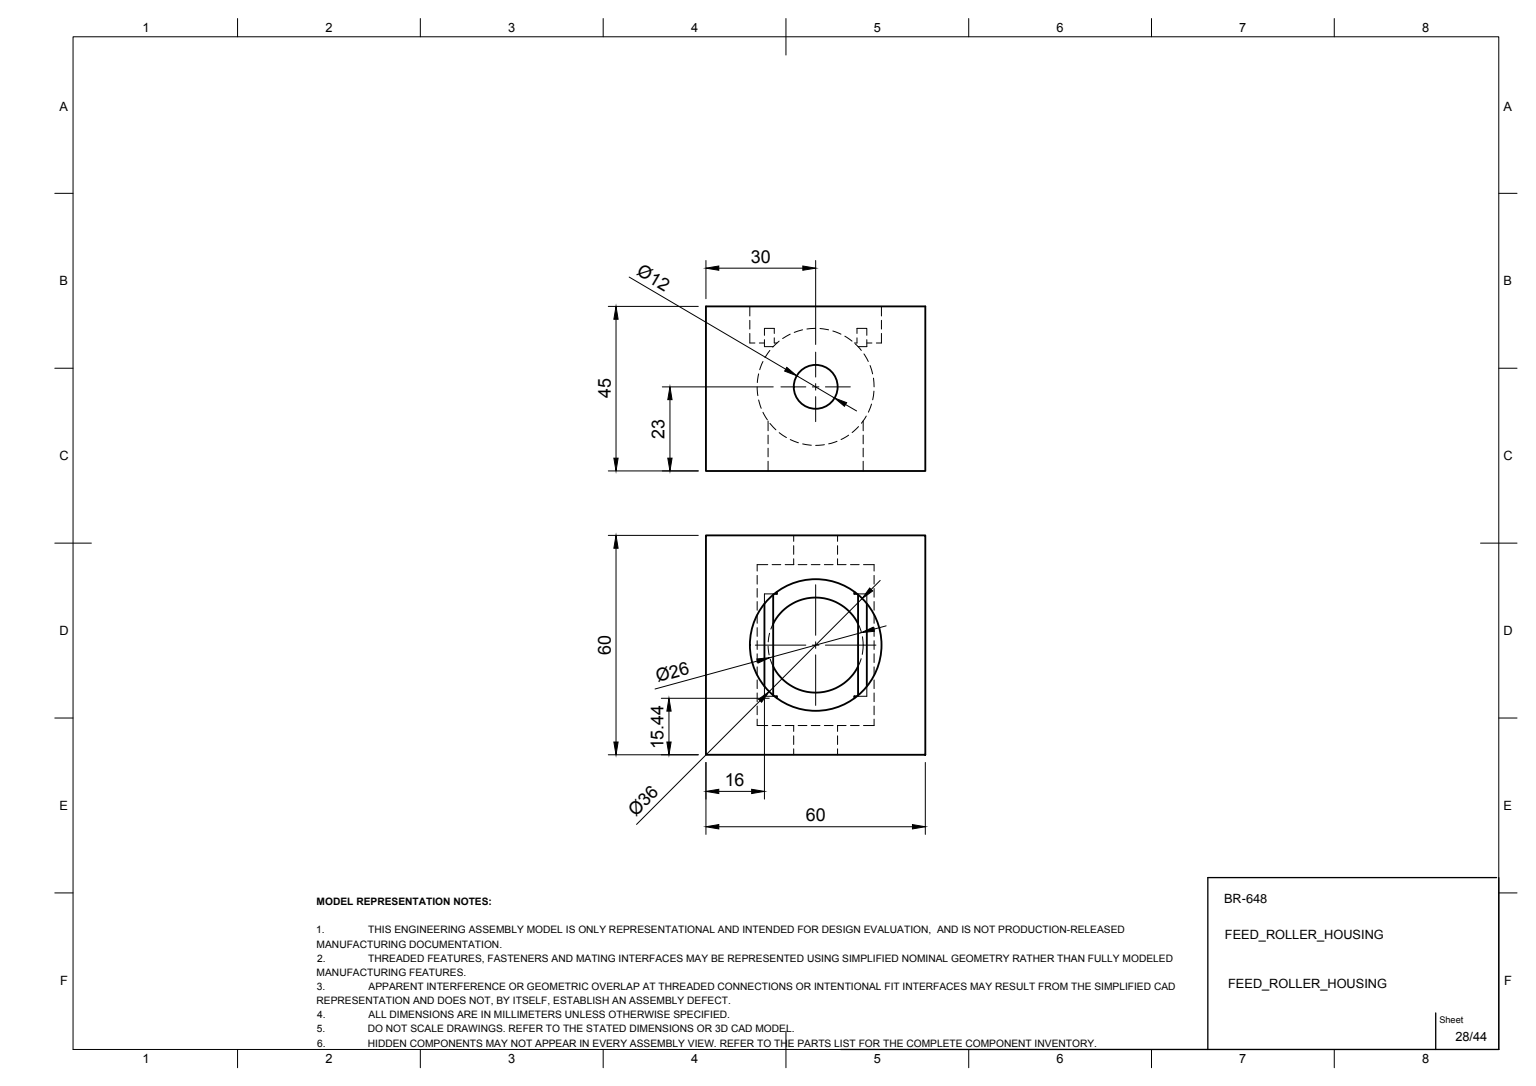
ISO-10303-21;
HEADER;
FILE_DESCRIPTION((''),'2;1');
FILE_NAME('FEED_ROLLER_HOUSING.step','2026-10-01T22:05:39-07:00',(''),(''),'','','');
FILE_SCHEMA (('AUTOMOTIVE_DESIGN { 1 0 10303 214 3 1 1 }'));
ENDSEC;
DATA;
#10=MECHANICAL_DESIGN_GEOMETRIC_PRESENTATION_REPRESENTATION('',(#626),#24628);
#542=SHAPE_REPRESENTATION_RELATIONSHIP('SRR','None',#24815,#584) ;
#584=ADVANCED_BREP_SHAPE_REPRESENTATION('',(#665),#24605) ;
#626=STYLED_ITEM('',(#25031),#665) ;
#665=MANIFOLD_SOLID_BREP('FEED_ROLLER_HOUSING',#13168) ;
#876=FACE_BOUND('',#4451,.T.) ;
#877=FACE_BOUND('',#4452,.T.) ;
#878=FACE_BOUND('',#4454,.T.) ;
#879=FACE_BOUND('',#4456,.T.) ;
#880=FACE_BOUND('',#4460,.T.) ;
#881=FACE_BOUND('',#4462,.T.) ;
#882=FACE_BOUND('',#4464,.T.) ;
#883=FACE_BOUND('',#4467,.T.) ;
#980=B_SPLINE_CURVE_WITH_KNOTS('',3,(#23034,#23035,#23036,#23037,#23038,
#23039,#23040,#23041,#23042,#23043,#23044,#23045,#23046,#23047,#23048,#23049,
#23050,#23051,#23052,#23053,#23054,#23055,#23056,#23057,#23058,#23059),
 .UNSPECIFIED.,.F.,.F.,(4,2,2,2,2,2,2,2,2,2,2,2,4),(0.,0.268031600880283,
0.536063201760566,1.07212640352113,1.58977454134265,1.84859861025342,2.10742267916418,
2.36624674807494,2.6250708169857,3.14271895480722,3.67878215656779,3.94681375744807,
4.21484535832835),.UNSPECIFIED.) ;
#981=B_SPLINE_CURVE_WITH_KNOTS('',3,(#23060,#23061,#23062,#23063,#23064,
#23065,#23066,#23067,#23068,#23069,#23070,#23071,#23072,#23073,#23074,#23075,
#23076,#23077,#23078,#23079,#23080,#23081,#23082,#23083,#23084,#23085),
 .UNSPECIFIED.,.F.,.F.,(4,2,2,2,2,2,2,2,2,2,2,2,4),(4.21484535832835,4.48287695920864,
4.75090856008892,5.28697176184949,5.80461989967101,6.06344396858177,6.32226803749253,
6.58109210640329,6.83991617531405,7.35756431313557,7.89362751489614,8.16165911577642,
8.42969071665671),.UNSPECIFIED.) ;
#982=B_SPLINE_CURVE_WITH_KNOTS('',3,(#23105,#23106,#23107,#23108,#23109,
#23110,#23111,#23112,#23113,#23114,#23115,#23116,#23117,#23118,#23119,#23120,
#23121,#23122),.UNSPECIFIED.,.F.,.F.,(4,2,2,2,2,2,2,2,4),(6.84192042814915,
7.05142392525706,7.37435159053249,7.69727925580792,8.02020692108334,8.34313458635877,
8.6660622516342,8.98898991690963,9.19849341401755),.UNSPECIFIED.) ;
#983=B_SPLINE_CURVE_WITH_KNOTS('',3,(#23124,#23125,#23126,#23127,#23128,
#23129,#23130,#23131,#23132,#23133,#23134,#23135,#23136,#23137,#23138,#23139,
#23140,#23141),.UNSPECIFIED.,.F.,.F.,(4,2,2,2,2,2,2,2,4),(1.49511581409358,
1.7046193112015,2.02754697647693,2.35047464175235,2.67340230702778,2.99632997230321,
3.31925763757864,3.64218530285406,3.85168879996198),.UNSPECIFIED.) ;
#1487=LINE('',#22927,#2323) ;
#1488=LINE('',#22929,#2324) ;
#1489=LINE('',#22931,#2325) ;
#1490=LINE('',#22933,#2326) ;
#1491=LINE('',#22935,#2327) ;
#1492=LINE('',#22937,#2328) ;
#1493=LINE('',#22939,#2329) ;
#1494=LINE('',#22940,#2330) ;
#1495=LINE('',#22944,#2331) ;
#1496=LINE('',#22946,#2332) ;
#1497=LINE('',#22948,#2333) ;
#1498=LINE('',#22949,#2334) ;
#1499=LINE('',#22954,#2335) ;
#1500=LINE('',#22956,#2336) ;
#1501=LINE('',#22958,#2337) ;
#1502=LINE('',#22959,#2338) ;
#1503=LINE('',#22964,#2339) ;
#1504=LINE('',#22966,#2340) ;
#1505=LINE('',#22968,#2341) ;
#1506=LINE('',#22969,#2342) ;
#1507=LINE('',#22973,#2343) ;
#1508=LINE('',#22974,#2344) ;
#1509=LINE('',#22976,#2345) ;
#1510=LINE('',#22979,#2346) ;
#1511=LINE('',#22983,#2347) ;
#1512=LINE('',#22989,#2348) ;
#1513=LINE('',#22993,#2349) ;
#1514=LINE('',#22996,#2350) ;
#1515=LINE('',#22997,#2351) ;
#1516=LINE('',#23000,#2352) ;
#1517=LINE('',#23002,#2353) ;
#1518=LINE('',#23006,#2354) ;
#1519=LINE('',#23008,#2355) ;
#1520=LINE('',#23009,#2356) ;
#1521=LINE('',#23012,#2357) ;
#1522=LINE('',#23017,#2358) ;
#1523=LINE('',#23025,#2359) ;
#1524=LINE('',#23032,#2360) ;
#1525=LINE('',#23090,#2361) ;
#1526=LINE('',#23096,#2362) ;
#1527=LINE('',#23102,#2363) ;
#1528=LINE('',#23123,#2364) ;
#1529=LINE('',#23148,#2365) ;
#1530=LINE('',#23153,#2366) ;
#1531=LINE('',#23155,#2367) ;
#1532=LINE('',#23157,#2368) ;
#1533=LINE('',#23158,#2369) ;
#1534=LINE('',#23162,#2370) ;
#1535=LINE('',#23164,#2371) ;
#1536=LINE('',#23166,#2372) ;
#1537=LINE('',#23167,#2373) ;
#1538=LINE('',#23169,#2374) ;
#1539=LINE('',#23170,#2375) ;
#1540=LINE('',#23172,#2376) ;
#1541=LINE('',#23174,#2377) ;
#2323=VECTOR('',#18344,1.) ;
#2324=VECTOR('',#18345,1.) ;
#2325=VECTOR('',#18346,1.) ;
#2326=VECTOR('',#18347,1.) ;
#2327=VECTOR('',#18348,1.) ;
#2328=VECTOR('',#18349,1.) ;
#2329=VECTOR('',#18350,1.) ;
#2330=VECTOR('',#18351,1.) ;
#2331=VECTOR('',#18354,1.) ;
#2332=VECTOR('',#18355,1.) ;
#2333=VECTOR('',#18356,1.) ;
#2334=VECTOR('',#18357,1.) ;
#2335=VECTOR('',#18362,1.) ;
#2336=VECTOR('',#18363,1.) ;
#2337=VECTOR('',#18364,1.) ;
#2338=VECTOR('',#18365,1.) ;
#2339=VECTOR('',#18370,1.) ;
#2340=VECTOR('',#18371,1.) ;
#2341=VECTOR('',#18372,1.) ;
#2342=VECTOR('',#18373,1.) ;
#2343=VECTOR('',#18376,1.) ;
#2344=VECTOR('',#18377,1.) ;
#2345=VECTOR('',#18378,1.) ;
#2346=VECTOR('',#18381,1.) ;
#2347=VECTOR('',#18386,1.) ;
#2348=VECTOR('',#18395,1.) ;
#2349=VECTOR('',#18400,1.) ;
#2350=VECTOR('',#18403,1.) ;
#2351=VECTOR('',#18404,1.) ;
#2352=VECTOR('',#18407,1.) ;
#2353=VECTOR('',#18408,1.) ;
#2354=VECTOR('',#18413,1.) ;
#2355=VECTOR('',#18414,1.) ;
#2356=VECTOR('',#18415,1.) ;
#2357=VECTOR('',#18418,1.) ;
#2358=VECTOR('',#18425,1.) ;
#2359=VECTOR('',#18436,1.) ;
#2360=VECTOR('',#18445,1.3) ;
#2361=VECTOR('',#18450,0.6) ;
#2362=VECTOR('',#18457,0.6) ;
#2363=VECTOR('',#18464,1.6) ;
#2364=VECTOR('',#18467,1.) ;
#2365=VECTOR('',#18478,1.8) ;
#2366=VECTOR('',#18483,1.) ;
#2367=VECTOR('',#18484,1.) ;
#2368=VECTOR('',#18485,1.) ;
#2369=VECTOR('',#18486,1.) ;
#2370=VECTOR('',#18489,1.) ;
#2371=VECTOR('',#18490,1.) ;
#2372=VECTOR('',#18491,1.) ;
#2373=VECTOR('',#18492,1.) ;
#2374=VECTOR('',#18495,1.) ;
#2375=VECTOR('',#18496,1.) ;
#2376=VECTOR('',#18499,1.) ;
#2377=VECTOR('',#18502,1.) ;
#2875=CYLINDRICAL_SURFACE('',#14916,1.3) ;
#2876=CYLINDRICAL_SURFACE('',#14918,0.6) ;
#2877=CYLINDRICAL_SURFACE('',#14921,0.6) ;
#2878=CYLINDRICAL_SURFACE('',#14924,1.6) ;
#2879=CYLINDRICAL_SURFACE('',#14931,1.8) ;
#3473=FACE_OUTER_BOUND('',#4430,.T.) ;
#3474=FACE_OUTER_BOUND('',#4431,.T.) ;
#3475=FACE_OUTER_BOUND('',#4432,.T.) ;
#3476=FACE_OUTER_BOUND('',#4433,.T.) ;
#3477=FACE_OUTER_BOUND('',#4434,.T.) ;
#3478=FACE_OUTER_BOUND('',#4435,.T.) ;
#3479=FACE_OUTER_BOUND('',#4436,.T.) ;
#3480=FACE_OUTER_BOUND('',#4437,.T.) ;
#3481=FACE_OUTER_BOUND('',#4438,.T.) ;
#3482=FACE_OUTER_BOUND('',#4439,.T.) ;
#3483=FACE_OUTER_BOUND('',#4440,.T.) ;
#3484=FACE_OUTER_BOUND('',#4441,.T.) ;
#3485=FACE_OUTER_BOUND('',#4442,.T.) ;
#3486=FACE_OUTER_BOUND('',#4443,.T.) ;
#3487=FACE_OUTER_BOUND('',#4444,.T.) ;
#3488=FACE_OUTER_BOUND('',#4445,.T.) ;
#3489=FACE_OUTER_BOUND('',#4446,.T.) ;
#3490=FACE_OUTER_BOUND('',#4447,.T.) ;
#3491=FACE_OUTER_BOUND('',#4448,.T.) ;
#3492=FACE_OUTER_BOUND('',#4449,.T.) ;
#3493=FACE_OUTER_BOUND('',#4450,.T.) ;
#3494=FACE_OUTER_BOUND('',#4453,.T.) ;
#3495=FACE_OUTER_BOUND('',#4455,.T.) ;
#3496=FACE_OUTER_BOUND('',#4457,.T.) ;
#3497=FACE_OUTER_BOUND('',#4458,.T.) ;
#3498=FACE_OUTER_BOUND('',#4459,.T.) ;
#3499=FACE_OUTER_BOUND('',#4461,.T.) ;
#3500=FACE_OUTER_BOUND('',#4463,.T.) ;
#3501=FACE_OUTER_BOUND('',#4465,.T.) ;
#3502=FACE_OUTER_BOUND('',#4466,.T.) ;
#3503=FACE_OUTER_BOUND('',#4468,.T.) ;
#4430=EDGE_LOOP('',(#10863,#10864,#10865,#10866,#10867,#10868,#10869,#10870)) ;
#4431=EDGE_LOOP('',(#10871,#10872,#10873,#10874)) ;
#4432=EDGE_LOOP('',(#10875,#10876,#10877,#10878,#10879,#10880)) ;
#4433=EDGE_LOOP('',(#10881,#10882,#10883,#10884,#10885,#10886)) ;
#4434=EDGE_LOOP('',(#10887,#10888,#10889,#10890,#10891,#10892)) ;
#4435=EDGE_LOOP('',(#10893,#10894,#10895)) ;
#4436=EDGE_LOOP('',(#10896,#10897,#10898)) ;
#4437=EDGE_LOOP('',(#10899,#10900,#10901)) ;
#4438=EDGE_LOOP('',(#10902,#10903,#10904)) ;
#4439=EDGE_LOOP('',(#10905,#10906,#10907,#10908)) ;
#4440=EDGE_LOOP('',(#10909,#10910,#10911,#10912,#10913,#10914)) ;
#4441=EDGE_LOOP('',(#10915,#10916,#10917,#10918,#10919,#10920,#10921,#10922)) ;
#4442=EDGE_LOOP('',(#10923,#10924,#10925)) ;
#4443=EDGE_LOOP('',(#10926,#10927,#10928)) ;
#4444=EDGE_LOOP('',(#10929,#10930,#10931)) ;
#4445=EDGE_LOOP('',(#10932,#10933,#10934)) ;
#4446=EDGE_LOOP('',(#10935,#10936)) ;
#4447=EDGE_LOOP('',(#10937,#10938,#10939,#10940,#10941)) ;
#4448=EDGE_LOOP('',(#10942,#10943,#10944,#10945)) ;
#4449=EDGE_LOOP('',(#10946,#10947,#10948,#10949)) ;
#4450=EDGE_LOOP('',(#10950,#10951,#10952,#10953)) ;
#4451=EDGE_LOOP('',(#10954,#10955,#10956,#10957,#10958,#10959,#10960,#10961,
#10962,#10963,#10964,#10965)) ;
#4452=EDGE_LOOP('',(#10966,#10967)) ;
#4453=EDGE_LOOP('',(#10968)) ;
#4454=EDGE_LOOP('',(#10969)) ;
#4455=EDGE_LOOP('',(#10970)) ;
#4456=EDGE_LOOP('',(#10971)) ;
#4457=EDGE_LOOP('',(#10972,#10973,#10974)) ;
#4458=EDGE_LOOP('',(#10975,#10976,#10977,#10978,#10979,#10980,#10981,#10982,
#10983,#10984,#10985,#10986,#10987,#10988,#10989,#10990,#10991,#10992,#10993,
#10994,#10995,#10996,#10997,#10998)) ;
#4459=EDGE_LOOP('',(#10999,#11000,#11001,#11002)) ;
#4460=EDGE_LOOP('',(#11003)) ;
#4461=EDGE_LOOP('',(#11004,#11005,#11006,#11007)) ;
#4462=EDGE_LOOP('',(#11008)) ;
#4463=EDGE_LOOP('',(#11009,#11010,#11011,#11012)) ;
#4464=EDGE_LOOP('',(#11013)) ;
#4465=EDGE_LOOP('',(#11014,#11015,#11016,#11017)) ;
#4466=EDGE_LOOP('',(#11018,#11019,#11020,#11021)) ;
#4467=EDGE_LOOP('',(#11022)) ;
#4468=EDGE_LOOP('',(#11023,#11024,#11025,#11026)) ;
#5348=CIRCLE('',#14888,1.6) ;
#5349=CIRCLE('',#14890,1.6) ;
#5350=CIRCLE('',#14892,1.6) ;
#5351=CIRCLE('',#14894,1.8) ;
#5352=CIRCLE('',#14896,1.8) ;
#5353=CIRCLE('',#14898,1.8) ;
#5354=CIRCLE('',#14900,1.8) ;
#5355=CIRCLE('',#14903,1.6) ;
#5356=CIRCLE('',#14906,1.8) ;
#5357=CIRCLE('',#14908,1.8) ;
#5358=CIRCLE('',#14910,1.8) ;
#5359=CIRCLE('',#14911,1.8) ;
#5360=CIRCLE('',#14913,1.8) ;
#5361=CIRCLE('',#14915,1.8) ;
#5362=CIRCLE('',#14917,1.3) ;
#5363=CIRCLE('',#14919,0.6) ;
#5364=CIRCLE('',#14920,0.6) ;
#5365=CIRCLE('',#14922,0.6) ;
#5366=CIRCLE('',#14923,0.6) ;
#5367=CIRCLE('',#14925,1.6) ;
#5368=CIRCLE('',#14926,1.6) ;
#5369=CIRCLE('',#14930,1.8) ;
#5370=CIRCLE('',#14932,1.8) ;
#6358=VERTEX_POINT('',#22925) ;
#6359=VERTEX_POINT('',#22926) ;
#6360=VERTEX_POINT('',#22928) ;
#6361=VERTEX_POINT('',#22930) ;
#6362=VERTEX_POINT('',#22932) ;
#6363=VERTEX_POINT('',#22934) ;
#6364=VERTEX_POINT('',#22936) ;
#6365=VERTEX_POINT('',#22938) ;
#6366=VERTEX_POINT('',#22942) ;
#6367=VERTEX_POINT('',#22943) ;
#6368=VERTEX_POINT('',#22945) ;
#6369=VERTEX_POINT('',#22947) ;
#6370=VERTEX_POINT('',#22951) ;
#6371=VERTEX_POINT('',#22953) ;
#6372=VERTEX_POINT('',#22955) ;
#6373=VERTEX_POINT('',#22957) ;
#6374=VERTEX_POINT('',#22961) ;
#6375=VERTEX_POINT('',#22963) ;
#6376=VERTEX_POINT('',#22965) ;
#6377=VERTEX_POINT('',#22967) ;
#6378=VERTEX_POINT('',#22971) ;
#6379=VERTEX_POINT('',#22972) ;
#6380=VERTEX_POINT('',#22975) ;
#6381=VERTEX_POINT('',#22977) ;
#6382=VERTEX_POINT('',#22981) ;
#6383=VERTEX_POINT('',#22987) ;
#6384=VERTEX_POINT('',#22991) ;
#6385=VERTEX_POINT('',#22995) ;
#6386=VERTEX_POINT('',#22999) ;
#6387=VERTEX_POINT('',#23001) ;
#6388=VERTEX_POINT('',#23005) ;
#6389=VERTEX_POINT('',#23007) ;
#6390=VERTEX_POINT('',#23011) ;
#6391=VERTEX_POINT('',#23015) ;
#6392=VERTEX_POINT('',#23019) ;
#6393=VERTEX_POINT('',#23023) ;
#6394=VERTEX_POINT('',#23029) ;
#6395=VERTEX_POINT('',#23031) ;
#6396=VERTEX_POINT('',#23033) ;
#6397=VERTEX_POINT('',#23087) ;
#6398=VERTEX_POINT('',#23089) ;
#6399=VERTEX_POINT('',#23093) ;
#6400=VERTEX_POINT('',#23095) ;
#6401=VERTEX_POINT('',#23099) ;
#6402=VERTEX_POINT('',#23101) ;
#6403=VERTEX_POINT('',#23104) ;
#6404=VERTEX_POINT('',#23147) ;
#6405=VERTEX_POINT('',#23151) ;
#6406=VERTEX_POINT('',#23152) ;
#6407=VERTEX_POINT('',#23154) ;
#6408=VERTEX_POINT('',#23156) ;
#6409=VERTEX_POINT('',#23160) ;
#6410=VERTEX_POINT('',#23161) ;
#6411=VERTEX_POINT('',#23163) ;
#6412=VERTEX_POINT('',#23165) ;
#7921=EDGE_CURVE('',#6358,#6359,#1487,.T.) ;
#7922=EDGE_CURVE('',#6358,#6360,#1488,.T.) ;
#7923=EDGE_CURVE('',#6360,#6361,#1489,.T.) ;
#7924=EDGE_CURVE('',#6361,#6362,#1490,.T.) ;
#7925=EDGE_CURVE('',#6363,#6362,#1491,.T.) ;
#7926=EDGE_CURVE('',#6363,#6364,#1492,.T.) ;
#7927=EDGE_CURVE('',#6365,#6364,#1493,.T.) ;
#7928=EDGE_CURVE('',#6359,#6365,#1494,.T.) ;
#7929=EDGE_CURVE('',#6366,#6367,#1495,.T.) ;
#7930=EDGE_CURVE('',#6368,#6366,#1496,.T.) ;
#7931=EDGE_CURVE('',#6369,#6368,#1497,.T.) ;
#7932=EDGE_CURVE('',#6367,#6369,#1498,.T.) ;
#7933=EDGE_CURVE('',#6370,#6366,#5348,.T.) ;
#7934=EDGE_CURVE('',#6371,#6370,#1499,.T.) ;
#7935=EDGE_CURVE('',#6372,#6371,#1500,.T.) ;
#7936=EDGE_CURVE('',#6372,#6373,#1501,.T.) ;
#7937=EDGE_CURVE('',#6373,#6368,#1502,.T.) ;
#7938=EDGE_CURVE('',#6367,#6374,#5349,.T.) ;
#7939=EDGE_CURVE('',#6375,#6369,#1503,.T.) ;
#7940=EDGE_CURVE('',#6375,#6376,#1504,.T.) ;
#7941=EDGE_CURVE('',#6377,#6376,#1505,.T.) ;
#7942=EDGE_CURVE('',#6374,#6377,#1506,.T.) ;
#7943=EDGE_CURVE('',#6378,#6379,#1507,.T.) ;
#7944=EDGE_CURVE('',#6378,#6363,#1508,.T.) ;
#7945=EDGE_CURVE('',#6362,#6380,#1509,.T.) ;
#7946=EDGE_CURVE('',#6381,#6380,#5350,.T.) ;
#7947=EDGE_CURVE('',#6379,#6381,#1510,.T.) ;
#7948=EDGE_CURVE('',#6376,#6382,#5351,.T.) ;
#7949=EDGE_CURVE('',#6382,#6375,#1511,.T.) ;
#7950=EDGE_CURVE('',#6364,#6378,#5352,.T.) ;
#7951=EDGE_CURVE('',#6383,#6372,#5353,.T.) ;
#7952=EDGE_CURVE('',#6373,#6383,#1512,.T.) ;
#7953=EDGE_CURVE('',#6384,#6358,#5354,.T.) ;
#7954=EDGE_CURVE('',#6360,#6384,#1513,.T.) ;
#7955=EDGE_CURVE('',#6380,#6385,#1514,.T.) ;
#7956=EDGE_CURVE('',#6385,#6361,#1515,.T.) ;
#7957=EDGE_CURVE('',#6386,#6384,#1516,.T.) ;
#7958=EDGE_CURVE('',#6387,#6386,#1517,.T.) ;
#7959=EDGE_CURVE('',#6385,#6387,#5355,.T.) ;
#7960=EDGE_CURVE('',#6388,#6383,#1518,.T.) ;
#7961=EDGE_CURVE('',#6389,#6388,#1519,.T.) ;
#7962=EDGE_CURVE('',#6382,#6389,#1520,.T.) ;
#7963=EDGE_CURVE('',#6381,#6390,#1521,.T.) ;
#7964=EDGE_CURVE('',#6379,#6390,#5356,.T.) ;
#7965=EDGE_CURVE('',#6391,#6386,#5357,.T.) ;
#7966=EDGE_CURVE('',#6391,#6387,#1522,.T.) ;
#7967=EDGE_CURVE('',#6392,#6365,#5358,.T.) ;
#7968=EDGE_CURVE('',#6359,#6392,#5359,.T.) ;
#7969=EDGE_CURVE('',#6393,#6377,#5360,.T.) ;
#7970=EDGE_CURVE('',#6393,#6374,#1523,.T.) ;
#7971=EDGE_CURVE('',#6389,#6388,#5361,.T.) ;
#7972=EDGE_CURVE('',#6394,#6394,#5362,.T.) ;
#7973=EDGE_CURVE('',#6394,#6395,#1524,.T.) ;
#7974=EDGE_CURVE('',#6396,#6395,#980,.T.) ;
#7975=EDGE_CURVE('',#6395,#6396,#981,.T.) ;
#7976=EDGE_CURVE('',#6397,#6397,#5363,.T.) ;
#7977=EDGE_CURVE('',#6397,#6398,#1525,.T.) ;
#7978=EDGE_CURVE('',#6398,#6398,#5364,.T.) ;
#7979=EDGE_CURVE('',#6399,#6399,#5365,.T.) ;
#7980=EDGE_CURVE('',#6399,#6400,#1526,.T.) ;
#7981=EDGE_CURVE('',#6400,#6400,#5366,.T.) ;
#7982=EDGE_CURVE('',#6401,#6401,#5367,.T.) ;
#7983=EDGE_CURVE('',#6401,#6402,#1527,.T.) ;
#7984=EDGE_CURVE('',#6402,#6402,#5368,.T.) ;
#7985=EDGE_CURVE('',#6403,#6391,#982,.T.) ;
#7986=EDGE_CURVE('',#6370,#6403,#1528,.T.) ;
#7987=EDGE_CURVE('',#6390,#6393,#983,.T.) ;
#7988=EDGE_CURVE('',#6371,#6403,#5369,.T.) ;
#7989=EDGE_CURVE('',#6392,#6404,#1529,.T.) ;
#7990=EDGE_CURVE('',#6404,#6404,#5370,.T.) ;
#7991=EDGE_CURVE('',#6405,#6406,#1530,.T.) ;
#7992=EDGE_CURVE('',#6406,#6407,#1531,.T.) ;
#7993=EDGE_CURVE('',#6407,#6408,#1532,.T.) ;
#7994=EDGE_CURVE('',#6408,#6405,#1533,.T.) ;
#7995=EDGE_CURVE('',#6409,#6410,#1534,.T.) ;
#7996=EDGE_CURVE('',#6410,#6411,#1535,.T.) ;
#7997=EDGE_CURVE('',#6411,#6412,#1536,.T.) ;
#7998=EDGE_CURVE('',#6412,#6409,#1537,.T.) ;
#7999=EDGE_CURVE('',#6408,#6411,#1538,.T.) ;
#8000=EDGE_CURVE('',#6405,#6410,#1539,.T.) ;
#8001=EDGE_CURVE('',#6407,#6412,#1540,.T.) ;
#8002=EDGE_CURVE('',#6406,#6409,#1541,.T.) ;
#10863=ORIENTED_EDGE('',*,*,#7921,.F.) ;
#10864=ORIENTED_EDGE('',*,*,#7922,.T.) ;
#10865=ORIENTED_EDGE('',*,*,#7923,.T.) ;
#10866=ORIENTED_EDGE('',*,*,#7924,.T.) ;
#10867=ORIENTED_EDGE('',*,*,#7925,.F.) ;
#10868=ORIENTED_EDGE('',*,*,#7926,.T.) ;
#10869=ORIENTED_EDGE('',*,*,#7927,.F.) ;
#10870=ORIENTED_EDGE('',*,*,#7928,.F.) ;
#10871=ORIENTED_EDGE('',*,*,#7929,.F.) ;
#10872=ORIENTED_EDGE('',*,*,#7930,.F.) ;
#10873=ORIENTED_EDGE('',*,*,#7931,.F.) ;
#10874=ORIENTED_EDGE('',*,*,#7932,.F.) ;
#10875=ORIENTED_EDGE('',*,*,#7933,.F.) ;
#10876=ORIENTED_EDGE('',*,*,#7934,.F.) ;
#10877=ORIENTED_EDGE('',*,*,#7935,.F.) ;
#10878=ORIENTED_EDGE('',*,*,#7936,.T.) ;
#10879=ORIENTED_EDGE('',*,*,#7937,.T.) ;
#10880=ORIENTED_EDGE('',*,*,#7930,.T.) ;
#10881=ORIENTED_EDGE('',*,*,#7938,.F.) ;
#10882=ORIENTED_EDGE('',*,*,#7932,.T.) ;
#10883=ORIENTED_EDGE('',*,*,#7939,.F.) ;
#10884=ORIENTED_EDGE('',*,*,#7940,.T.) ;
#10885=ORIENTED_EDGE('',*,*,#7941,.F.) ;
#10886=ORIENTED_EDGE('',*,*,#7942,.F.) ;
#10887=ORIENTED_EDGE('',*,*,#7943,.F.) ;
#10888=ORIENTED_EDGE('',*,*,#7944,.T.) ;
#10889=ORIENTED_EDGE('',*,*,#7925,.T.) ;
#10890=ORIENTED_EDGE('',*,*,#7945,.T.) ;
#10891=ORIENTED_EDGE('',*,*,#7946,.F.) ;
#10892=ORIENTED_EDGE('',*,*,#7947,.F.) ;
#10893=ORIENTED_EDGE('',*,*,#7948,.F.) ;
#10894=ORIENTED_EDGE('',*,*,#7940,.F.) ;
#10895=ORIENTED_EDGE('',*,*,#7949,.F.) ;
#10896=ORIENTED_EDGE('',*,*,#7950,.F.) ;
#10897=ORIENTED_EDGE('',*,*,#7926,.F.) ;
#10898=ORIENTED_EDGE('',*,*,#7944,.F.) ;
#10899=ORIENTED_EDGE('',*,*,#7951,.F.) ;
#10900=ORIENTED_EDGE('',*,*,#7952,.F.) ;
#10901=ORIENTED_EDGE('',*,*,#7936,.F.) ;
#10902=ORIENTED_EDGE('',*,*,#7953,.F.) ;
#10903=ORIENTED_EDGE('',*,*,#7954,.F.) ;
#10904=ORIENTED_EDGE('',*,*,#7922,.F.) ;
#10905=ORIENTED_EDGE('',*,*,#7955,.F.) ;
#10906=ORIENTED_EDGE('',*,*,#7945,.F.) ;
#10907=ORIENTED_EDGE('',*,*,#7924,.F.) ;
#10908=ORIENTED_EDGE('',*,*,#7956,.F.) ;
#10909=ORIENTED_EDGE('',*,*,#7957,.F.) ;
#10910=ORIENTED_EDGE('',*,*,#7958,.F.) ;
#10911=ORIENTED_EDGE('',*,*,#7959,.F.) ;
#10912=ORIENTED_EDGE('',*,*,#7956,.T.) ;
#10913=ORIENTED_EDGE('',*,*,#7923,.F.) ;
#10914=ORIENTED_EDGE('',*,*,#7954,.T.) ;
#10915=ORIENTED_EDGE('',*,*,#7960,.F.) ;
#10916=ORIENTED_EDGE('',*,*,#7961,.F.) ;
#10917=ORIENTED_EDGE('',*,*,#7962,.F.) ;
#10918=ORIENTED_EDGE('',*,*,#7949,.T.) ;
#10919=ORIENTED_EDGE('',*,*,#7939,.T.) ;
#10920=ORIENTED_EDGE('',*,*,#7931,.T.) ;
#10921=ORIENTED_EDGE('',*,*,#7937,.F.) ;
#10922=ORIENTED_EDGE('',*,*,#7952,.T.) ;
#10923=ORIENTED_EDGE('',*,*,#7947,.T.) ;
#10924=ORIENTED_EDGE('',*,*,#7963,.T.) ;
#10925=ORIENTED_EDGE('',*,*,#7964,.F.) ;
#10926=ORIENTED_EDGE('',*,*,#7958,.T.) ;
#10927=ORIENTED_EDGE('',*,*,#7965,.F.) ;
#10928=ORIENTED_EDGE('',*,*,#7966,.T.) ;
#10929=ORIENTED_EDGE('',*,*,#7928,.T.) ;
#10930=ORIENTED_EDGE('',*,*,#7967,.F.) ;
#10931=ORIENTED_EDGE('',*,*,#7968,.F.) ;
#10932=ORIENTED_EDGE('',*,*,#7942,.T.) ;
#10933=ORIENTED_EDGE('',*,*,#7969,.F.) ;
#10934=ORIENTED_EDGE('',*,*,#7970,.T.) ;
#10935=ORIENTED_EDGE('',*,*,#7961,.T.) ;
#10936=ORIENTED_EDGE('',*,*,#7971,.F.) ;
#10937=ORIENTED_EDGE('',*,*,#7972,.F.) ;
#10938=ORIENTED_EDGE('',*,*,#7973,.T.) ;
#10939=ORIENTED_EDGE('',*,*,#7974,.F.) ;
#10940=ORIENTED_EDGE('',*,*,#7975,.F.) ;
#10941=ORIENTED_EDGE('',*,*,#7973,.F.) ;
#10942=ORIENTED_EDGE('',*,*,#7976,.F.) ;
#10943=ORIENTED_EDGE('',*,*,#7977,.T.) ;
#10944=ORIENTED_EDGE('',*,*,#7978,.F.) ;
#10945=ORIENTED_EDGE('',*,*,#7977,.F.) ;
#10946=ORIENTED_EDGE('',*,*,#7979,.F.) ;
#10947=ORIENTED_EDGE('',*,*,#7980,.T.) ;
#10948=ORIENTED_EDGE('',*,*,#7981,.F.) ;
#10949=ORIENTED_EDGE('',*,*,#7980,.F.) ;
#10950=ORIENTED_EDGE('',*,*,#7982,.T.) ;
#10951=ORIENTED_EDGE('',*,*,#7983,.T.) ;
#10952=ORIENTED_EDGE('',*,*,#7984,.T.) ;
#10953=ORIENTED_EDGE('',*,*,#7983,.F.) ;
#10954=ORIENTED_EDGE('',*,*,#7959,.T.) ;
#10955=ORIENTED_EDGE('',*,*,#7966,.F.) ;
#10956=ORIENTED_EDGE('',*,*,#7985,.F.) ;
#10957=ORIENTED_EDGE('',*,*,#7986,.F.) ;
#10958=ORIENTED_EDGE('',*,*,#7933,.T.) ;
#10959=ORIENTED_EDGE('',*,*,#7929,.T.) ;
#10960=ORIENTED_EDGE('',*,*,#7938,.T.) ;
#10961=ORIENTED_EDGE('',*,*,#7970,.F.) ;
#10962=ORIENTED_EDGE('',*,*,#7987,.F.) ;
#10963=ORIENTED_EDGE('',*,*,#7963,.F.) ;
#10964=ORIENTED_EDGE('',*,*,#7946,.T.) ;
#10965=ORIENTED_EDGE('',*,*,#7955,.T.) ;
#10966=ORIENTED_EDGE('',*,*,#7974,.T.) ;
#10967=ORIENTED_EDGE('',*,*,#7975,.T.) ;
#10968=ORIENTED_EDGE('',*,*,#7982,.F.) ;
#10969=ORIENTED_EDGE('',*,*,#7981,.T.) ;
#10970=ORIENTED_EDGE('',*,*,#7984,.F.) ;
#10971=ORIENTED_EDGE('',*,*,#7976,.T.) ;
#10972=ORIENTED_EDGE('',*,*,#7934,.T.) ;
#10973=ORIENTED_EDGE('',*,*,#7986,.T.) ;
#10974=ORIENTED_EDGE('',*,*,#7988,.F.) ;
#10975=ORIENTED_EDGE('',*,*,#7921,.T.) ;
#10976=ORIENTED_EDGE('',*,*,#7968,.T.) ;
#10977=ORIENTED_EDGE('',*,*,#7989,.T.) ;
#10978=ORIENTED_EDGE('',*,*,#7990,.F.) ;
#10979=ORIENTED_EDGE('',*,*,#7989,.F.) ;
#10980=ORIENTED_EDGE('',*,*,#7967,.T.) ;
#10981=ORIENTED_EDGE('',*,*,#7927,.T.) ;
#10982=ORIENTED_EDGE('',*,*,#7950,.T.) ;
#10983=ORIENTED_EDGE('',*,*,#7943,.T.) ;
#10984=ORIENTED_EDGE('',*,*,#7964,.T.) ;
#10985=ORIENTED_EDGE('',*,*,#7987,.T.) ;
#10986=ORIENTED_EDGE('',*,*,#7969,.T.) ;
#10987=ORIENTED_EDGE('',*,*,#7941,.T.) ;
#10988=ORIENTED_EDGE('',*,*,#7948,.T.) ;
#10989=ORIENTED_EDGE('',*,*,#7962,.T.) ;
#10990=ORIENTED_EDGE('',*,*,#7971,.T.) ;
#10991=ORIENTED_EDGE('',*,*,#7960,.T.) ;
#10992=ORIENTED_EDGE('',*,*,#7951,.T.) ;
#10993=ORIENTED_EDGE('',*,*,#7935,.T.) ;
#10994=ORIENTED_EDGE('',*,*,#7988,.T.) ;
#10995=ORIENTED_EDGE('',*,*,#7985,.T.) ;
#10996=ORIENTED_EDGE('',*,*,#7965,.T.) ;
#10997=ORIENTED_EDGE('',*,*,#7957,.T.) ;
#10998=ORIENTED_EDGE('',*,*,#7953,.T.) ;
#10999=ORIENTED_EDGE('',*,*,#7991,.T.) ;
#11000=ORIENTED_EDGE('',*,*,#7992,.T.) ;
#11001=ORIENTED_EDGE('',*,*,#7993,.T.) ;
#11002=ORIENTED_EDGE('',*,*,#7994,.T.) ;
#11003=ORIENTED_EDGE('',*,*,#7990,.T.) ;
#11004=ORIENTED_EDGE('',*,*,#7995,.T.) ;
#11005=ORIENTED_EDGE('',*,*,#7996,.T.) ;
#11006=ORIENTED_EDGE('',*,*,#7997,.T.) ;
#11007=ORIENTED_EDGE('',*,*,#7998,.T.) ;
#11008=ORIENTED_EDGE('',*,*,#7972,.T.) ;
#11009=ORIENTED_EDGE('',*,*,#7999,.T.) ;
#11010=ORIENTED_EDGE('',*,*,#7996,.F.) ;
#11011=ORIENTED_EDGE('',*,*,#8000,.F.) ;
#11012=ORIENTED_EDGE('',*,*,#7994,.F.) ;
#11013=ORIENTED_EDGE('',*,*,#7979,.T.) ;
#11014=ORIENTED_EDGE('',*,*,#8001,.T.) ;
#11015=ORIENTED_EDGE('',*,*,#7997,.F.) ;
#11016=ORIENTED_EDGE('',*,*,#7999,.F.) ;
#11017=ORIENTED_EDGE('',*,*,#7993,.F.) ;
#11018=ORIENTED_EDGE('',*,*,#8002,.T.) ;
#11019=ORIENTED_EDGE('',*,*,#7998,.F.) ;
#11020=ORIENTED_EDGE('',*,*,#8001,.F.) ;
#11021=ORIENTED_EDGE('',*,*,#7992,.F.) ;
#11022=ORIENTED_EDGE('',*,*,#7978,.T.) ;
#11023=ORIENTED_EDGE('',*,*,#8000,.T.) ;
#11024=ORIENTED_EDGE('',*,*,#7995,.F.) ;
#11025=ORIENTED_EDGE('',*,*,#8002,.F.) ;
#11026=ORIENTED_EDGE('',*,*,#7991,.F.) ;
#12183=PLANE('',#14885) ;
#12184=PLANE('',#14886) ;
#12185=PLANE('',#14887) ;
#12186=PLANE('',#14889) ;
#12187=PLANE('',#14891) ;
#12188=PLANE('',#14893) ;
#12189=PLANE('',#14895) ;
#12190=PLANE('',#14897) ;
#12191=PLANE('',#14899) ;
#12192=PLANE('',#14901) ;
#12193=PLANE('',#14902) ;
#12194=PLANE('',#14904) ;
#12195=PLANE('',#14905) ;
#12196=PLANE('',#14907) ;
#12197=PLANE('',#14909) ;
#12198=PLANE('',#14912) ;
#12199=PLANE('',#14914) ;
#12200=PLANE('',#14927) ;
#12201=PLANE('',#14928) ;
#12202=PLANE('',#14929) ;
#12203=PLANE('',#14933) ;
#12204=PLANE('',#14934) ;
#12205=PLANE('',#14935) ;
#12206=PLANE('',#14936) ;
#12207=PLANE('',#14937) ;
#12208=PLANE('',#14938) ;
#12868=ADVANCED_FACE('',(#3473),#12183,.T.) ;
#12869=ADVANCED_FACE('',(#3474),#12184,.T.) ;
#12870=ADVANCED_FACE('',(#3475),#12185,.T.) ;
#12871=ADVANCED_FACE('',(#3476),#12186,.T.) ;
#12872=ADVANCED_FACE('',(#3477),#12187,.T.) ;
#12873=ADVANCED_FACE('',(#3478),#12188,.F.) ;
#12874=ADVANCED_FACE('',(#3479),#12189,.F.) ;
#12875=ADVANCED_FACE('',(#3480),#12190,.F.) ;
#12876=ADVANCED_FACE('',(#3481),#12191,.F.) ;
#12877=ADVANCED_FACE('',(#3482),#12192,.T.) ;
#12878=ADVANCED_FACE('',(#3483),#12193,.T.) ;
#12879=ADVANCED_FACE('',(#3484),#12194,.T.) ;
#12880=ADVANCED_FACE('',(#3485),#12195,.F.) ;
#12881=ADVANCED_FACE('',(#3486),#12196,.F.) ;
#12882=ADVANCED_FACE('',(#3487),#12197,.F.) ;
#12883=ADVANCED_FACE('',(#3488),#12198,.F.) ;
#12884=ADVANCED_FACE('',(#3489),#12199,.F.) ;
#12885=ADVANCED_FACE('',(#3490),#2875,.F.) ;
#12886=ADVANCED_FACE('',(#3491),#2876,.F.) ;
#12887=ADVANCED_FACE('',(#3492),#2877,.F.) ;
#12888=ADVANCED_FACE('',(#3493,#876,#877),#2878,.F.) ;
#12889=ADVANCED_FACE('',(#3494,#878),#12200,.F.) ;
#12890=ADVANCED_FACE('',(#3495,#879),#12201,.F.) ;
#12891=ADVANCED_FACE('',(#3496),#12202,.F.) ;
#12892=ADVANCED_FACE('',(#3497),#2879,.F.) ;
#12893=ADVANCED_FACE('',(#3498,#880),#12203,.T.) ;
#12894=ADVANCED_FACE('',(#3499,#881),#12204,.F.) ;
#12895=ADVANCED_FACE('',(#3500,#882),#12205,.F.) ;
#12896=ADVANCED_FACE('',(#3501),#12206,.F.) ;
#12897=ADVANCED_FACE('',(#3502,#883),#12207,.F.) ;
#12898=ADVANCED_FACE('',(#3503),#12208,.F.) ;
#13168=CLOSED_SHELL('',(#12868,#12869,#12870,#12871,#12872,#12873,#12874,
#12875,#12876,#12877,#12878,#12879,#12880,#12881,#12882,#12883,#12884,#12885,
#12886,#12887,#12888,#12889,#12890,#12891,#12892,#12893,#12894,#12895,#12896,
#12897,#12898)) ;
#14884=AXIS2_PLACEMENT_3D('',#22923,#18340,#18341) ;
#14885=AXIS2_PLACEMENT_3D('',#22924,#18342,#18343) ;
#14886=AXIS2_PLACEMENT_3D('',#22941,#18352,#18353) ;
#14887=AXIS2_PLACEMENT_3D('',#22950,#18358,#18359) ;
#14888=AXIS2_PLACEMENT_3D('',#22952,#18360,#18361) ;
#14889=AXIS2_PLACEMENT_3D('',#22960,#18366,#18367) ;
#14890=AXIS2_PLACEMENT_3D('',#22962,#18368,#18369) ;
#14891=AXIS2_PLACEMENT_3D('',#22970,#18374,#18375) ;
#14892=AXIS2_PLACEMENT_3D('',#22978,#18379,#18380) ;
#14893=AXIS2_PLACEMENT_3D('',#22980,#18382,#18383) ;
#14894=AXIS2_PLACEMENT_3D('',#22982,#18384,#18385) ;
#14895=AXIS2_PLACEMENT_3D('',#22984,#18387,#18388) ;
#14896=AXIS2_PLACEMENT_3D('',#22985,#18389,#18390) ;
#14897=AXIS2_PLACEMENT_3D('',#22986,#18391,#18392) ;
#14898=AXIS2_PLACEMENT_3D('',#22988,#18393,#18394) ;
#14899=AXIS2_PLACEMENT_3D('',#22990,#18396,#18397) ;
#14900=AXIS2_PLACEMENT_3D('',#22992,#18398,#18399) ;
#14901=AXIS2_PLACEMENT_3D('',#22994,#18401,#18402) ;
#14902=AXIS2_PLACEMENT_3D('',#22998,#18405,#18406) ;
#14903=AXIS2_PLACEMENT_3D('',#23003,#18409,#18410) ;
#14904=AXIS2_PLACEMENT_3D('',#23004,#18411,#18412) ;
#14905=AXIS2_PLACEMENT_3D('',#23010,#18416,#18417) ;
#14906=AXIS2_PLACEMENT_3D('',#23013,#18419,#18420) ;
#14907=AXIS2_PLACEMENT_3D('',#23014,#18421,#18422) ;
#14908=AXIS2_PLACEMENT_3D('',#23016,#18423,#18424) ;
#14909=AXIS2_PLACEMENT_3D('',#23018,#18426,#18427) ;
#14910=AXIS2_PLACEMENT_3D('',#23020,#18428,#18429) ;
#14911=AXIS2_PLACEMENT_3D('',#23021,#18430,#18431) ;
#14912=AXIS2_PLACEMENT_3D('',#23022,#18432,#18433) ;
#14913=AXIS2_PLACEMENT_3D('',#23024,#18434,#18435) ;
#14914=AXIS2_PLACEMENT_3D('',#23026,#18437,#18438) ;
#14915=AXIS2_PLACEMENT_3D('',#23027,#18439,#18440) ;
#14916=AXIS2_PLACEMENT_3D('',#23028,#18441,#18442) ;
#14917=AXIS2_PLACEMENT_3D('',#23030,#18443,#18444) ;
#14918=AXIS2_PLACEMENT_3D('',#23086,#18446,#18447) ;
#14919=AXIS2_PLACEMENT_3D('',#23088,#18448,#18449) ;
#14920=AXIS2_PLACEMENT_3D('',#23091,#18451,#18452) ;
#14921=AXIS2_PLACEMENT_3D('',#23092,#18453,#18454) ;
#14922=AXIS2_PLACEMENT_3D('',#23094,#18455,#18456) ;
#14923=AXIS2_PLACEMENT_3D('',#23097,#18458,#18459) ;
#14924=AXIS2_PLACEMENT_3D('',#23098,#18460,#18461) ;
#14925=AXIS2_PLACEMENT_3D('',#23100,#18462,#18463) ;
#14926=AXIS2_PLACEMENT_3D('',#23103,#18465,#18466) ;
#14927=AXIS2_PLACEMENT_3D('',#23142,#18468,#18469) ;
#14928=AXIS2_PLACEMENT_3D('',#23143,#18470,#18471) ;
#14929=AXIS2_PLACEMENT_3D('',#23144,#18472,#18473) ;
#14930=AXIS2_PLACEMENT_3D('',#23145,#18474,#18475) ;
#14931=AXIS2_PLACEMENT_3D('',#23146,#18476,#18477) ;
#14932=AXIS2_PLACEMENT_3D('',#23149,#18479,#18480) ;
#14933=AXIS2_PLACEMENT_3D('',#23150,#18481,#18482) ;
#14934=AXIS2_PLACEMENT_3D('',#23159,#18487,#18488) ;
#14935=AXIS2_PLACEMENT_3D('',#23168,#18493,#18494) ;
#14936=AXIS2_PLACEMENT_3D('',#23171,#18497,#18498) ;
#14937=AXIS2_PLACEMENT_3D('',#23173,#18500,#18501) ;
#14938=AXIS2_PLACEMENT_3D('',#23175,#18503,#18504) ;
#18340=DIRECTION('axis',(0.,0.,1.)) ;
#18341=DIRECTION('refdir',(1.,0.,0.)) ;
#18342=DIRECTION('center_axis',(1.,0.,0.)) ;
#18343=DIRECTION('ref_axis',(0.,0.,-1.)) ;
#18344=DIRECTION('',(0.,0.,-1.)) ;
#18345=DIRECTION('',(0.,-1.,0.)) ;
#18346=DIRECTION('',(0.,0.,-1.)) ;
#18347=DIRECTION('',(0.,1.,0.)) ;
#18348=DIRECTION('',(0.,0.,-1.)) ;
#18349=DIRECTION('',(0.,-1.,0.)) ;
#18350=DIRECTION('',(0.,0.,1.)) ;
#18351=DIRECTION('',(0.,1.,0.)) ;
#18352=DIRECTION('center_axis',(0.,0.,1.)) ;
#18353=DIRECTION('ref_axis',(1.,0.,0.)) ;
#18354=DIRECTION('',(0.,1.,0.)) ;
#18355=DIRECTION('',(-1.,0.,0.)) ;
#18356=DIRECTION('',(0.,-1.,0.)) ;
#18357=DIRECTION('',(1.,0.,0.)) ;
#18358=DIRECTION('center_axis',(0.,1.,0.)) ;
#18359=DIRECTION('ref_axis',(0.,0.,1.)) ;
#18360=DIRECTION('center_axis',(0.,1.,0.)) ;
#18361=DIRECTION('ref_axis',(1.,0.,0.)) ;
#18362=DIRECTION('',(-1.,0.,0.)) ;
#18363=DIRECTION('',(0.,0.,-1.)) ;
#18364=DIRECTION('',(1.,0.,0.)) ;
#18365=DIRECTION('',(0.,0.,-1.)) ;
#18366=DIRECTION('center_axis',(0.,-1.,0.)) ;
#18367=DIRECTION('ref_axis',(0.,0.,-1.)) ;
#18368=DIRECTION('center_axis',(0.,-1.,0.)) ;
#18369=DIRECTION('ref_axis',(1.,0.,0.)) ;
#18370=DIRECTION('',(0.,0.,-1.)) ;
#18371=DIRECTION('',(-1.,0.,0.)) ;
#18372=DIRECTION('',(0.,0.,1.)) ;
#18373=DIRECTION('',(1.,0.,0.)) ;
#18374=DIRECTION('center_axis',(0.,-1.,0.)) ;
#18375=DIRECTION('ref_axis',(0.,0.,-1.)) ;
#18376=DIRECTION('',(0.,0.,-1.)) ;
#18377=DIRECTION('',(-1.,0.,0.)) ;
#18378=DIRECTION('',(1.,0.,0.)) ;
#18379=DIRECTION('center_axis',(0.,-1.,0.)) ;
#18380=DIRECTION('ref_axis',(1.,0.,0.)) ;
#18381=DIRECTION('',(1.,0.,0.)) ;
#18382=DIRECTION('center_axis',(0.,0.,1.)) ;
#18383=DIRECTION('ref_axis',(1.,0.,0.)) ;
#18384=DIRECTION('center_axis',(0.,0.,-1.)) ;
#18385=DIRECTION('ref_axis',(1.,0.,0.)) ;
#18386=DIRECTION('',(0.,1.,0.)) ;
#18387=DIRECTION('center_axis',(0.,0.,1.)) ;
#18388=DIRECTION('ref_axis',(1.,0.,0.)) ;
#18389=DIRECTION('center_axis',(0.,0.,-1.)) ;
#18390=DIRECTION('ref_axis',(1.,0.,0.)) ;
#18391=DIRECTION('center_axis',(0.,0.,1.)) ;
#18392=DIRECTION('ref_axis',(1.,0.,0.)) ;
#18393=DIRECTION('center_axis',(0.,0.,-1.)) ;
#18394=DIRECTION('ref_axis',(1.,0.,0.)) ;
#18395=DIRECTION('',(0.,1.,0.)) ;
#18396=DIRECTION('center_axis',(0.,0.,1.)) ;
#18397=DIRECTION('ref_axis',(1.,0.,0.)) ;
#18398=DIRECTION('center_axis',(0.,0.,-1.)) ;
#18399=DIRECTION('ref_axis',(1.,0.,0.)) ;
#18400=DIRECTION('',(1.,0.,0.)) ;
#18401=DIRECTION('center_axis',(0.,0.,1.)) ;
#18402=DIRECTION('ref_axis',(1.,0.,0.)) ;
#18403=DIRECTION('',(0.,-1.,0.)) ;
#18404=DIRECTION('',(-1.,0.,0.)) ;
#18405=DIRECTION('center_axis',(0.,1.,0.)) ;
#18406=DIRECTION('ref_axis',(0.,0.,1.)) ;
#18407=DIRECTION('',(0.,0.,1.)) ;
#18408=DIRECTION('',(-1.,0.,0.)) ;
#18409=DIRECTION('center_axis',(0.,1.,0.)) ;
#18410=DIRECTION('ref_axis',(1.,0.,0.)) ;
#18411=DIRECTION('center_axis',(-1.,0.,0.)) ;
#18412=DIRECTION('ref_axis',(0.,0.,1.)) ;
#18413=DIRECTION('',(0.,0.,1.)) ;
#18414=DIRECTION('',(0.,-1.,0.)) ;
#18415=DIRECTION('',(0.,0.,-1.)) ;
#18416=DIRECTION('center_axis',(0.,0.,-1.)) ;
#18417=DIRECTION('ref_axis',(-1.,0.,0.)) ;
#18418=DIRECTION('',(0.,1.,0.)) ;
#18419=DIRECTION('center_axis',(0.,0.,-1.)) ;
#18420=DIRECTION('ref_axis',(1.,0.,0.)) ;
#18421=DIRECTION('center_axis',(0.,0.,-1.)) ;
#18422=DIRECTION('ref_axis',(-1.,0.,0.)) ;
#18423=DIRECTION('center_axis',(0.,0.,-1.)) ;
#18424=DIRECTION('ref_axis',(1.,0.,0.)) ;
#18425=DIRECTION('',(0.,1.,0.)) ;
#18426=DIRECTION('center_axis',(0.,0.,-1.)) ;
#18427=DIRECTION('ref_axis',(-1.,0.,0.)) ;
#18428=DIRECTION('center_axis',(0.,0.,-1.)) ;
#18429=DIRECTION('ref_axis',(1.,0.,0.)) ;
#18430=DIRECTION('center_axis',(0.,0.,-1.)) ;
#18431=DIRECTION('ref_axis',(1.,0.,0.)) ;
#18432=DIRECTION('center_axis',(0.,0.,-1.)) ;
#18433=DIRECTION('ref_axis',(-1.,0.,0.)) ;
#18434=DIRECTION('center_axis',(0.,0.,-1.)) ;
#18435=DIRECTION('ref_axis',(1.,0.,0.)) ;
#18436=DIRECTION('',(0.,-1.,0.)) ;
#18437=DIRECTION('center_axis',(0.,0.,-1.)) ;
#18438=DIRECTION('ref_axis',(-1.,0.,0.)) ;
#18439=DIRECTION('center_axis',(0.,0.,-1.)) ;
#18440=DIRECTION('ref_axis',(1.,0.,0.)) ;
#18441=DIRECTION('center_axis',(0.,0.,1.)) ;
#18442=DIRECTION('ref_axis',(1.,0.,0.)) ;
#18443=DIRECTION('center_axis',(0.,0.,1.)) ;
#18444=DIRECTION('ref_axis',(1.,0.,0.)) ;
#18445=DIRECTION('',(0.,0.,1.)) ;
#18446=DIRECTION('center_axis',(0.,1.,0.)) ;
#18447=DIRECTION('ref_axis',(1.,0.,0.)) ;
#18448=DIRECTION('center_axis',(0.,1.,0.)) ;
#18449=DIRECTION('ref_axis',(1.,0.,0.)) ;
#18450=DIRECTION('',(0.,1.,0.)) ;
#18451=DIRECTION('center_axis',(0.,-1.,0.)) ;
#18452=DIRECTION('ref_axis',(1.,0.,0.)) ;
#18453=DIRECTION('center_axis',(0.,1.,0.)) ;
#18454=DIRECTION('ref_axis',(1.,0.,0.)) ;
#18455=DIRECTION('center_axis',(0.,1.,0.)) ;
#18456=DIRECTION('ref_axis',(1.,0.,0.)) ;
#18457=DIRECTION('',(0.,1.,0.)) ;
#18458=DIRECTION('center_axis',(0.,-1.,0.)) ;
#18459=DIRECTION('ref_axis',(1.,0.,0.)) ;
#18460=DIRECTION('center_axis',(0.,1.,0.)) ;
#18461=DIRECTION('ref_axis',(1.,0.,0.)) ;
#18462=DIRECTION('center_axis',(0.,-1.,0.)) ;
#18463=DIRECTION('ref_axis',(1.,0.,0.)) ;
#18464=DIRECTION('',(0.,1.,0.)) ;
#18465=DIRECTION('center_axis',(0.,1.,0.)) ;
#18466=DIRECTION('ref_axis',(1.,0.,0.)) ;
#18467=DIRECTION('',(0.,-1.,0.)) ;
#18468=DIRECTION('center_axis',(0.,-1.,0.)) ;
#18469=DIRECTION('ref_axis',(-1.,0.,0.)) ;
#18470=DIRECTION('center_axis',(0.,1.,0.)) ;
#18471=DIRECTION('ref_axis',(1.,0.,0.)) ;
#18472=DIRECTION('center_axis',(0.,0.,-1.)) ;
#18473=DIRECTION('ref_axis',(-1.,0.,0.)) ;
#18474=DIRECTION('center_axis',(0.,0.,-1.)) ;
#18475=DIRECTION('ref_axis',(1.,0.,0.)) ;
#18476=DIRECTION('center_axis',(0.,0.,1.)) ;
#18477=DIRECTION('ref_axis',(1.,0.,0.)) ;
#18478=DIRECTION('',(0.,0.,1.)) ;
#18479=DIRECTION('center_axis',(0.,0.,-1.)) ;
#18480=DIRECTION('ref_axis',(1.,0.,0.)) ;
#18481=DIRECTION('center_axis',(0.,0.,1.)) ;
#18482=DIRECTION('ref_axis',(1.,0.,0.)) ;
#18483=DIRECTION('',(0.,1.,0.)) ;
#18484=DIRECTION('',(-1.,0.,0.)) ;
#18485=DIRECTION('',(0.,-1.,0.)) ;
#18486=DIRECTION('',(1.,0.,0.)) ;
#18487=DIRECTION('center_axis',(0.,0.,1.)) ;
#18488=DIRECTION('ref_axis',(1.,0.,0.)) ;
#18489=DIRECTION('',(0.,-1.,0.)) ;
#18490=DIRECTION('',(-1.,0.,0.)) ;
#18491=DIRECTION('',(0.,1.,0.)) ;
#18492=DIRECTION('',(1.,0.,0.)) ;
#18493=DIRECTION('center_axis',(0.,1.,0.)) ;
#18494=DIRECTION('ref_axis',(0.,0.,1.)) ;
#18495=DIRECTION('',(0.,0.,-1.)) ;
#18496=DIRECTION('',(0.,0.,-1.)) ;
#18497=DIRECTION('center_axis',(1.,0.,0.)) ;
#18498=DIRECTION('ref_axis',(0.,0.,-1.)) ;
#18499=DIRECTION('',(0.,0.,-1.)) ;
#18500=DIRECTION('center_axis',(0.,-1.,0.)) ;
#18501=DIRECTION('ref_axis',(0.,0.,-1.)) ;
#18502=DIRECTION('',(0.,0.,-1.)) ;
#18503=DIRECTION('center_axis',(-1.,0.,0.)) ;
#18504=DIRECTION('ref_axis',(0.,0.,1.)) ;
#22923=CARTESIAN_POINT('',(0.,0.,0.)) ;
#22924=CARTESIAN_POINT('Origin',(-24.4,-1.8,-0.85)) ;
#22925=CARTESIAN_POINT('',(-24.4,-2.93137084989848,-0.6)) ;
#22926=CARTESIAN_POINT('',(-24.4,-2.93137084989848,-1.)) ;
#22927=CARTESIAN_POINT('',(-24.4,-2.93137084989848,-0.45)) ;
#22928=CARTESIAN_POINT('',(-24.4,-3.2,-0.6)) ;
#22929=CARTESIAN_POINT('',(-24.4,-1.8,-0.6)) ;
#22930=CARTESIAN_POINT('',(-24.4,-3.2,-1.1)) ;
#22931=CARTESIAN_POINT('',(-24.4,-3.2,-0.85)) ;
#22932=CARTESIAN_POINT('',(-24.4,-0.4,-1.1)) ;
#22933=CARTESIAN_POINT('',(-24.4,-1.8,-1.1)) ;
#22934=CARTESIAN_POINT('',(-24.4,-0.4,-0.6)) ;
#22935=CARTESIAN_POINT('',(-24.4,-0.4,-0.85)) ;
#22936=CARTESIAN_POINT('',(-24.4,-0.668629150101522,-0.6)) ;
#22937=CARTESIAN_POINT('',(-24.4,-1.8,-0.6)) ;
#22938=CARTESIAN_POINT('',(-24.4,-0.668629150101522,-1.)) ;
#22939=CARTESIAN_POINT('',(-24.4,-0.668629150101522,-0.45)) ;
#22940=CARTESIAN_POINT('',(-24.4,-1.8,-1.)) ;
#22941=CARTESIAN_POINT('Origin',(-23.,-1.8,-1.1)) ;
#22942=CARTESIAN_POINT('',(-21.8381049961378,-3.2,-1.1)) ;
#22943=CARTESIAN_POINT('',(-21.8381049961378,-0.4,-1.1)) ;
#22944=CARTESIAN_POINT('',(-21.8381049961378,-1.8,-1.1)) ;
#22945=CARTESIAN_POINT('',(-21.6,-3.2,-1.1)) ;
#22946=CARTESIAN_POINT('',(-23.,-3.2,-1.1)) ;
#22947=CARTESIAN_POINT('',(-21.6,-0.4,-1.1)) ;
#22948=CARTESIAN_POINT('',(-21.6,-1.8,-1.1)) ;
#22949=CARTESIAN_POINT('',(-23.,-0.4,-1.1)) ;
#22950=CARTESIAN_POINT('Origin',(-23.,-3.2,-0.85)) ;
#22951=CARTESIAN_POINT('',(-21.9416994755742,-3.2,-1.)) ;
#22952=CARTESIAN_POINT('Origin',(-23.,-3.2,-2.2)) ;
#22953=CARTESIAN_POINT('',(-21.8686291501015,-3.2,-1.)) ;
#22954=CARTESIAN_POINT('',(-23.,-3.2,-1.)) ;
#22955=CARTESIAN_POINT('',(-21.8686291501015,-3.2,-0.6)) ;
#22956=CARTESIAN_POINT('',(-21.8686291501015,-3.2,-0.45)) ;
#22957=CARTESIAN_POINT('',(-21.6,-3.2,-0.6)) ;
#22958=CARTESIAN_POINT('',(-23.,-3.2,-0.6)) ;
#22959=CARTESIAN_POINT('',(-21.6,-3.2,-0.85)) ;
#22960=CARTESIAN_POINT('Origin',(-23.,-0.4,-0.85)) ;
#22961=CARTESIAN_POINT('',(-21.9416994755742,-0.4,-1.)) ;
#22962=CARTESIAN_POINT('Origin',(-23.,-0.4,-2.2)) ;
#22963=CARTESIAN_POINT('',(-21.6,-0.4,-0.6)) ;
#22964=CARTESIAN_POINT('',(-21.6,-0.4,-0.85)) ;
#22965=CARTESIAN_POINT('',(-21.8686291501015,-0.4,-0.6)) ;
#22966=CARTESIAN_POINT('',(-23.,-0.4,-0.6)) ;
#22967=CARTESIAN_POINT('',(-21.8686291501015,-0.4,-1.)) ;
#22968=CARTESIAN_POINT('',(-21.8686291501015,-0.4,-0.45)) ;
#22969=CARTESIAN_POINT('',(-23.,-0.4,-1.)) ;
#22970=CARTESIAN_POINT('Origin',(-23.,-0.4,-0.85)) ;
#22971=CARTESIAN_POINT('',(-24.1313708498985,-0.4,-0.6)) ;
#22972=CARTESIAN_POINT('',(-24.1313708498985,-0.4,-1.)) ;
#22973=CARTESIAN_POINT('',(-24.1313708498985,-0.4,-0.45)) ;
#22974=CARTESIAN_POINT('',(-23.,-0.4,-0.6)) ;
#22975=CARTESIAN_POINT('',(-24.1618950038622,-0.4,-1.1)) ;
#22976=CARTESIAN_POINT('',(-23.,-0.4,-1.1)) ;
#22977=CARTESIAN_POINT('',(-24.0583005244258,-0.4,-1.)) ;
#22978=CARTESIAN_POINT('Origin',(-23.,-0.4,-2.2)) ;
#22979=CARTESIAN_POINT('',(-23.,-0.4,-1.)) ;
#22980=CARTESIAN_POINT('Origin',(-23.,-1.8,-0.6)) ;
#22981=CARTESIAN_POINT('',(-21.6,-0.668629150101522,-0.6)) ;
#22982=CARTESIAN_POINT('Origin',(-23.,-1.8,-0.6)) ;
#22983=CARTESIAN_POINT('',(-21.6,-1.8,-0.6)) ;
#22984=CARTESIAN_POINT('Origin',(-23.,-1.8,-0.6)) ;
#22985=CARTESIAN_POINT('Origin',(-23.,-1.8,-0.6)) ;
#22986=CARTESIAN_POINT('Origin',(-23.,-1.8,-0.6)) ;
#22987=CARTESIAN_POINT('',(-21.6,-2.93137084989848,-0.6)) ;
#22988=CARTESIAN_POINT('Origin',(-23.,-1.8,-0.6)) ;
#22989=CARTESIAN_POINT('',(-21.6,-1.8,-0.6)) ;
#22990=CARTESIAN_POINT('Origin',(-23.,-1.8,-0.6)) ;
#22991=CARTESIAN_POINT('',(-24.1313708498985,-3.2,-0.6)) ;
#22992=CARTESIAN_POINT('Origin',(-23.,-1.8,-0.6)) ;
#22993=CARTESIAN_POINT('',(-23.,-3.2,-0.6)) ;
#22994=CARTESIAN_POINT('Origin',(-23.,-1.8,-1.1)) ;
#22995=CARTESIAN_POINT('',(-24.1618950038622,-3.2,-1.1)) ;
#22996=CARTESIAN_POINT('',(-24.1618950038622,-1.8,-1.1)) ;
#22997=CARTESIAN_POINT('',(-23.,-3.2,-1.1)) ;
#22998=CARTESIAN_POINT('Origin',(-23.,-3.2,-0.85)) ;
#22999=CARTESIAN_POINT('',(-24.1313708498985,-3.2,-1.)) ;
#23000=CARTESIAN_POINT('',(-24.1313708498985,-3.2,-0.45)) ;
#23001=CARTESIAN_POINT('',(-24.0583005244258,-3.2,-1.)) ;
#23002=CARTESIAN_POINT('',(-23.,-3.2,-1.)) ;
#23003=CARTESIAN_POINT('Origin',(-23.,-3.2,-2.2)) ;
#23004=CARTESIAN_POINT('Origin',(-21.6,-1.8,-0.85)) ;
#23005=CARTESIAN_POINT('',(-21.6,-2.93137084989848,-1.)) ;
#23006=CARTESIAN_POINT('',(-21.6,-2.93137084989848,-0.45)) ;
#23007=CARTESIAN_POINT('',(-21.6,-0.668629150101522,-1.)) ;
#23008=CARTESIAN_POINT('',(-21.6,-1.8,-1.)) ;
#23009=CARTESIAN_POINT('',(-21.6,-0.668629150101522,-0.45)) ;
#23010=CARTESIAN_POINT('Origin',(-23.,-1.8,-1.)) ;
#23011=CARTESIAN_POINT('',(-24.0583005244258,-0.343978022143896,-1.)) ;
#23012=CARTESIAN_POINT('',(-24.0583005244258,-1.8,-1.)) ;
#23013=CARTESIAN_POINT('Origin',(-23.,-1.8,-1.)) ;
#23014=CARTESIAN_POINT('Origin',(-23.,-1.8,-1.)) ;
#23015=CARTESIAN_POINT('',(-24.0583005244258,-3.2560219778561,-1.)) ;
#23016=CARTESIAN_POINT('Origin',(-23.,-1.8,-1.)) ;
#23017=CARTESIAN_POINT('',(-24.0583005244258,-1.8,-1.)) ;
#23018=CARTESIAN_POINT('Origin',(-23.,-1.8,-1.)) ;
#23019=CARTESIAN_POINT('',(-24.8,-1.8,-1.)) ;
#23020=CARTESIAN_POINT('Origin',(-23.,-1.8,-1.)) ;
#23021=CARTESIAN_POINT('Origin',(-23.,-1.8,-1.)) ;
#23022=CARTESIAN_POINT('Origin',(-23.,-1.8,-1.)) ;
#23023=CARTESIAN_POINT('',(-21.9416994755742,-0.343978022143896,-1.)) ;
#23024=CARTESIAN_POINT('Origin',(-23.,-1.8,-1.)) ;
#23025=CARTESIAN_POINT('',(-21.9416994755742,-1.8,-1.)) ;
#23026=CARTESIAN_POINT('Origin',(-23.,-1.8,-1.)) ;
#23027=CARTESIAN_POINT('Origin',(-23.,-1.8,-1.)) ;
#23028=CARTESIAN_POINT('Origin',(-23.,-1.8,-3.4)) ;
#23029=CARTESIAN_POINT('',(-24.3,-1.8,-4.5)) ;
#23030=CARTESIAN_POINT('Origin',(-23.,-1.8,-4.5)) ;
#23031=CARTESIAN_POINT('',(-24.3,-1.8,-3.13273790530888)) ;
#23032=CARTESIAN_POINT('',(-24.3,-1.8,-3.4)) ;
#23033=CARTESIAN_POINT('',(-21.7,-1.8,-3.13273790530888)) ;
#23034=CARTESIAN_POINT('Ctrl Pts',(-21.7,-1.8,-3.13273790530888)) ;
#23035=CARTESIAN_POINT('Ctrl Pts',(-21.7,-1.88934386696009,-3.13273790530888)) ;
#23036=CARTESIAN_POINT('Ctrl Pts',(-21.7092429454133,-1.97758308210185,
-3.14593464346712)) ;
#23037=CARTESIAN_POINT('Ctrl Pts',(-21.7444789059789,-2.14821877213838,
-3.19222623476834)) ;
#23038=CARTESIAN_POINT('Ctrl Pts',(-21.7704660290006,-2.23068508647083,
-3.22506776421433)) ;
#23039=CARTESIAN_POINT('Ctrl Pts',(-21.8704353089628,-2.46562551307362,
-3.33760910141692)) ;
#23040=CARTESIAN_POINT('Ctrl Pts',(-21.9675840369442,-2.60606166802919,
-3.43013719509726)) ;
#23041=CARTESIAN_POINT('Ctrl Pts',(-22.1900504239759,-2.82852805506094,
-3.58629392075118)) ;
#23042=CARTESIAN_POINT('Ctrl Pts',(-22.3305352921443,-2.92774057937871,
-3.66289157340511)) ;
#23043=CARTESIAN_POINT('Ctrl Pts',(-22.5694255964999,-3.02967523999069,
-3.74326420954647)) ;
#23044=CARTESIAN_POINT('Ctrl Pts',(-22.6537071359882,-3.05610474843748,
-3.76450988863227)) ;
#23045=CARTESIAN_POINT('Ctrl Pts',(-22.8258541681822,-3.09127499629695,
-3.79288517120475)) ;
#23046=CARTESIAN_POINT('Ctrl Pts',(-22.9137253103631,-3.1,-3.8)) ;
#23047=CARTESIAN_POINT('Ctrl Pts',(-23.0862746896369,-3.1,-3.8)) ;
#23048=CARTESIAN_POINT('Ctrl Pts',(-23.1741458318178,-3.09127499629695,
-3.79288517120475)) ;
#23049=CARTESIAN_POINT('Ctrl Pts',(-23.3462928640118,-3.05610474843748,
-3.76450988863227)) ;
#23050=CARTESIAN_POINT('Ctrl Pts',(-23.4305744035001,-3.02967523999069,
-3.74326420954647)) ;
#23051=CARTESIAN_POINT('Ctrl Pts',(-23.6694647078557,-2.92774057937871,
-3.66289157340511)) ;
#23052=CARTESIAN_POINT('Ctrl Pts',(-23.8099495760241,-2.82852805506094,
-3.58629392075118)) ;
#23053=CARTESIAN_POINT('Ctrl Pts',(-24.0324159630558,-2.60606166802919,
-3.43013719509726)) ;
#23054=CARTESIAN_POINT('Ctrl Pts',(-24.1295646910372,-2.46562551307362,
-3.33760910141692)) ;
#23055=CARTESIAN_POINT('Ctrl Pts',(-24.2295339709994,-2.23068508647083,
-3.22506776421433)) ;
#23056=CARTESIAN_POINT('Ctrl Pts',(-24.2555210940211,-2.14821877213838,
-3.19222623476834)) ;
#23057=CARTESIAN_POINT('Ctrl Pts',(-24.2907570545867,-1.97758308210185,
-3.14593464346712)) ;
#23058=CARTESIAN_POINT('Ctrl Pts',(-24.3,-1.88934386696009,-3.13273790530888)) ;
#23059=CARTESIAN_POINT('Ctrl Pts',(-24.3,-1.8,-3.13273790530888)) ;
#23060=CARTESIAN_POINT('Ctrl Pts',(-24.3,-1.8,-3.13273790530888)) ;
#23061=CARTESIAN_POINT('Ctrl Pts',(-24.3,-1.71065613303991,-3.13273790530888)) ;
#23062=CARTESIAN_POINT('Ctrl Pts',(-24.2907570545867,-1.62241691789815,
-3.14593464346712)) ;
#23063=CARTESIAN_POINT('Ctrl Pts',(-24.2555210940211,-1.45178122786162,
-3.19222623476834)) ;
#23064=CARTESIAN_POINT('Ctrl Pts',(-24.2295339709994,-1.36931491352917,
-3.22506776421433)) ;
#23065=CARTESIAN_POINT('Ctrl Pts',(-24.1295646910372,-1.13437448692638,
-3.33760910141692)) ;
#23066=CARTESIAN_POINT('Ctrl Pts',(-24.0324159630558,-0.993938331970815,
-3.43013719509726)) ;
#23067=CARTESIAN_POINT('Ctrl Pts',(-23.8099495760241,-0.771471944939062,
-3.58629392075118)) ;
#23068=CARTESIAN_POINT('Ctrl Pts',(-23.6694647078557,-0.672259420621293,
-3.66289157340511)) ;
#23069=CARTESIAN_POINT('Ctrl Pts',(-23.4305744035001,-0.57032476000931,
-3.74326420954647)) ;
#23070=CARTESIAN_POINT('Ctrl Pts',(-23.3462928640118,-0.543895251562523,
-3.76450988863227)) ;
#23071=CARTESIAN_POINT('Ctrl Pts',(-23.1741458318178,-0.508725003703049,
-3.79288517120475)) ;
#23072=CARTESIAN_POINT('Ctrl Pts',(-23.0862746896369,-0.5,-3.8)) ;
#23073=CARTESIAN_POINT('Ctrl Pts',(-22.9137253103631,-0.5,-3.8)) ;
#23074=CARTESIAN_POINT('Ctrl Pts',(-22.8258541681822,-0.508725003703048,
-3.79288517120475)) ;
#23075=CARTESIAN_POINT('Ctrl Pts',(-22.6537071359882,-0.543895251562522,
-3.76450988863227)) ;
#23076=CARTESIAN_POINT('Ctrl Pts',(-22.5694255964999,-0.57032476000931,
-3.74326420954647)) ;
#23077=CARTESIAN_POINT('Ctrl Pts',(-22.3305352921443,-0.672259420621292,
-3.66289157340511)) ;
#23078=CARTESIAN_POINT('Ctrl Pts',(-22.1900504239759,-0.771471944939062,
-3.58629392075118)) ;
#23079=CARTESIAN_POINT('Ctrl Pts',(-21.9675840369442,-0.993938331970815,
-3.43013719509727)) ;
#23080=CARTESIAN_POINT('Ctrl Pts',(-21.8704353089629,-1.13437448692638,
-3.33760910141692)) ;
#23081=CARTESIAN_POINT('Ctrl Pts',(-21.7704660290006,-1.36931491352917,
-3.22506776421433)) ;
#23082=CARTESIAN_POINT('Ctrl Pts',(-21.7444789059789,-1.45178122786162,
-3.19222623476834)) ;
#23083=CARTESIAN_POINT('Ctrl Pts',(-21.7092429454133,-1.62241691789815,
-3.14593464346712)) ;
#23084=CARTESIAN_POINT('Ctrl Pts',(-21.7,-1.71065613303991,-3.13273790530888)) ;
#23085=CARTESIAN_POINT('Ctrl Pts',(-21.7,-1.8,-3.13273790530888)) ;
#23086=CARTESIAN_POINT('Origin',(-23.,0.85,-2.2)) ;
#23087=CARTESIAN_POINT('',(-23.6,0.4,-2.2)) ;
#23088=CARTESIAN_POINT('Origin',(-23.,0.4,-2.2)) ;
#23089=CARTESIAN_POINT('',(-23.6,1.2,-2.2)) ;
#23090=CARTESIAN_POINT('',(-23.6,0.85,-2.2)) ;
#23091=CARTESIAN_POINT('Origin',(-23.,1.2,-2.2)) ;
#23092=CARTESIAN_POINT('Origin',(-23.,-4.45,-2.2)) ;
#23093=CARTESIAN_POINT('',(-23.6,-4.8,-2.2)) ;
#23094=CARTESIAN_POINT('Origin',(-23.,-4.8,-2.2)) ;
#23095=CARTESIAN_POINT('',(-23.6,-4.,-2.2)) ;
#23096=CARTESIAN_POINT('',(-23.6,-4.45,-2.2)) ;
#23097=CARTESIAN_POINT('Origin',(-23.,-4.,-2.2)) ;
#23098=CARTESIAN_POINT('Origin',(-23.,-1.8,-2.2)) ;
#23099=CARTESIAN_POINT('',(-24.6,-4.,-2.2)) ;
#23100=CARTESIAN_POINT('Origin',(-23.,-4.,-2.2)) ;
#23101=CARTESIAN_POINT('',(-24.6,0.4,-2.2)) ;
#23102=CARTESIAN_POINT('',(-24.6,-1.8,-2.2)) ;
#23103=CARTESIAN_POINT('Origin',(-23.,0.4,-2.2)) ;
#23104=CARTESIAN_POINT('',(-21.9416994755742,-3.2560219778561,-1.)) ;
#23105=CARTESIAN_POINT('Ctrl Pts',(-21.9416994755742,-3.2560219778561,-1.)) ;
#23106=CARTESIAN_POINT('Ctrl Pts',(-21.9887809898529,-3.29024288386558,
-0.958478007290045)) ;
#23107=CARTESIAN_POINT('Ctrl Pts',(-22.0397004336828,-3.32373989107144,
-0.918526128699895)) ;
#23108=CARTESIAN_POINT('Ctrl Pts',(-22.1778690387736,-3.40421498216876,
-0.823614470242593)) ;
#23109=CARTESIAN_POINT('Ctrl Pts',(-22.2699364549541,-3.44861974206838,
-0.772284437575066)) ;
#23110=CARTESIAN_POINT('Ctrl Pts',(-22.4658004734772,-3.522083283395,-0.688049104156577)) ;
#23111=CARTESIAN_POINT('Ctrl Pts',(-22.5698376966291,-3.55120288441554,
-0.655067419610661)) ;
#23112=CARTESIAN_POINT('Ctrl Pts',(-22.7831124317021,-3.59017064340857,
-0.611033018569699)) ;
#23113=CARTESIAN_POINT('Ctrl Pts',(-22.8923574449082,-3.6,-0.6)) ;
#23114=CARTESIAN_POINT('Ctrl Pts',(-23.1076425550918,-3.6,-0.6)) ;
#23115=CARTESIAN_POINT('Ctrl Pts',(-23.2168875682979,-3.59017064340857,
-0.611033018569699)) ;
#23116=CARTESIAN_POINT('Ctrl Pts',(-23.4301623033709,-3.55120288441554,
-0.655067419610661)) ;
#23117=CARTESIAN_POINT('Ctrl Pts',(-23.5341995265228,-3.522083283395,-0.688049104156577)) ;
#23118=CARTESIAN_POINT('Ctrl Pts',(-23.7300635450459,-3.44861974206838,
-0.772284437575065)) ;
#23119=CARTESIAN_POINT('Ctrl Pts',(-23.8221309612264,-3.40421498216876,
-0.823614470242593)) ;
#23120=CARTESIAN_POINT('Ctrl Pts',(-23.9602995663172,-3.32373989107144,
-0.918526128699897)) ;
#23121=CARTESIAN_POINT('Ctrl Pts',(-24.0112190101471,-3.29024288386558,
-0.958478007290042)) ;
#23122=CARTESIAN_POINT('Ctrl Pts',(-24.0583005244258,-3.2560219778561,-1.)) ;
#23123=CARTESIAN_POINT('',(-21.9416994755742,-1.8,-1.)) ;
#23124=CARTESIAN_POINT('Ctrl Pts',(-24.0583005244258,-0.343978022143899,
-1.)) ;
#23125=CARTESIAN_POINT('Ctrl Pts',(-24.0112190101471,-0.309757116134422,
-0.958478007290048)) ;
#23126=CARTESIAN_POINT('Ctrl Pts',(-23.9602995663172,-0.276260108928558,
-0.918526128699897)) ;
#23127=CARTESIAN_POINT('Ctrl Pts',(-23.8221309612264,-0.195785017831241,
-0.823614470242595)) ;
#23128=CARTESIAN_POINT('Ctrl Pts',(-23.7300635450459,-0.151380257931619,
-0.772284437575069)) ;
#23129=CARTESIAN_POINT('Ctrl Pts',(-23.5341995265228,-0.0779167166050007,
-0.688049104156581)) ;
#23130=CARTESIAN_POINT('Ctrl Pts',(-23.4301623033709,-0.0487971155844649,
-0.655067419610662)) ;
#23131=CARTESIAN_POINT('Ctrl Pts',(-23.2168875682979,-0.00982935659143309,
-0.611033018569699)) ;
#23132=CARTESIAN_POINT('Ctrl Pts',(-23.1076425550918,0.,-0.6)) ;
#23133=CARTESIAN_POINT('Ctrl Pts',(-22.8923574449082,0.,-0.6)) ;
#23134=CARTESIAN_POINT('Ctrl Pts',(-22.7831124317021,-0.00982935659143327,
-0.611033018569699)) ;
#23135=CARTESIAN_POINT('Ctrl Pts',(-22.5698376966291,-0.048797115584464,
-0.655067419610661)) ;
#23136=CARTESIAN_POINT('Ctrl Pts',(-22.4658004734772,-0.0779167166049992,
-0.688049104156577)) ;
#23137=CARTESIAN_POINT('Ctrl Pts',(-22.2699364549541,-0.151380257931616,
-0.772284437575065)) ;
#23138=CARTESIAN_POINT('Ctrl Pts',(-22.1778690387736,-0.195785017831238,
-0.823614470242593)) ;
#23139=CARTESIAN_POINT('Ctrl Pts',(-22.0397004336828,-0.276260108928556,
-0.918526128699896)) ;
#23140=CARTESIAN_POINT('Ctrl Pts',(-21.9887809898529,-0.309757116134418,
-0.958478007290042)) ;
#23141=CARTESIAN_POINT('Ctrl Pts',(-21.9416994755742,-0.343978022143895,
-0.999999999999998)) ;
#23142=CARTESIAN_POINT('Origin',(-23.,-4.,-2.2)) ;
#23143=CARTESIAN_POINT('Origin',(-23.,0.4,-2.2)) ;
#23144=CARTESIAN_POINT('Origin',(-23.,-1.8,-1.)) ;
#23145=CARTESIAN_POINT('Origin',(-23.,-1.8,-1.)) ;
#23146=CARTESIAN_POINT('Origin',(-23.,-1.8,-0.45)) ;
#23147=CARTESIAN_POINT('',(-24.8,-1.8,0.)) ;
#23148=CARTESIAN_POINT('',(-24.8,-1.8,-0.45)) ;
#23149=CARTESIAN_POINT('Origin',(-23.,-1.8,0.)) ;
#23150=CARTESIAN_POINT('Origin',(-23.,-1.8,0.)) ;
#23151=CARTESIAN_POINT('',(-20.,-4.8,0.)) ;
#23152=CARTESIAN_POINT('',(-20.,1.2,0.)) ;
#23153=CARTESIAN_POINT('',(-20.,-1.8,0.)) ;
#23154=CARTESIAN_POINT('',(-26.,1.2,0.)) ;
#23155=CARTESIAN_POINT('',(-23.,1.2,0.)) ;
#23156=CARTESIAN_POINT('',(-26.,-4.8,0.)) ;
#23157=CARTESIAN_POINT('',(-26.,-1.8,0.)) ;
#23158=CARTESIAN_POINT('',(-23.,-4.8,0.)) ;
#23159=CARTESIAN_POINT('Origin',(-23.,-1.8,-4.5)) ;
#23160=CARTESIAN_POINT('',(-20.,1.2,-4.5)) ;
#23161=CARTESIAN_POINT('',(-20.,-4.8,-4.5)) ;
#23162=CARTESIAN_POINT('',(-20.,-1.8,-4.5)) ;
#23163=CARTESIAN_POINT('',(-26.,-4.8,-4.5)) ;
#23164=CARTESIAN_POINT('',(-23.,-4.8,-4.5)) ;
#23165=CARTESIAN_POINT('',(-26.,1.2,-4.5)) ;
#23166=CARTESIAN_POINT('',(-26.,-1.8,-4.5)) ;
#23167=CARTESIAN_POINT('',(-23.,1.2,-4.5)) ;
#23168=CARTESIAN_POINT('Origin',(-23.,-4.8,-2.25)) ;
#23169=CARTESIAN_POINT('',(-26.,-4.8,-2.25)) ;
#23170=CARTESIAN_POINT('',(-20.,-4.8,-2.25)) ;
#23171=CARTESIAN_POINT('Origin',(-26.,-1.8,-2.25)) ;
#23172=CARTESIAN_POINT('',(-26.,1.2,-2.25)) ;
#23173=CARTESIAN_POINT('Origin',(-23.,1.2,-2.25)) ;
#23174=CARTESIAN_POINT('',(-20.,1.2,-2.25)) ;
#23175=CARTESIAN_POINT('Origin',(-20.,-1.8,-2.25)) ;
#24557=UNCERTAINTY_MEASURE_WITH_UNIT(LENGTH_MEASURE(0.001),#24629,
'DISTANCE_ACCURACY_VALUE',
'Maximum model space distance between geometric entities at asserted c
onnectivities') ;
#24580=UNCERTAINTY_MEASURE_WITH_UNIT(LENGTH_MEASURE(0.001),#24629,
'DISTANCE_ACCURACY_VALUE',
'Maximum model space distance between geometric entities at asserted c
onnectivities') ;
#24605=(
GEOMETRIC_REPRESENTATION_CONTEXT(3)
GLOBAL_UNCERTAINTY_ASSIGNED_CONTEXT((#24557))
GLOBAL_UNIT_ASSIGNED_CONTEXT((#24629,#24631,#24632))
REPRESENTATION_CONTEXT('','3D')
) ;
#24628=(
GEOMETRIC_REPRESENTATION_CONTEXT(3)
GLOBAL_UNCERTAINTY_ASSIGNED_CONTEXT((#24580))
GLOBAL_UNIT_ASSIGNED_CONTEXT((#24629,#24631,#24632))
REPRESENTATION_CONTEXT('','3D')
) ;
#24629=(
LENGTH_UNIT()
NAMED_UNIT(*)
SI_UNIT(.CENTI.,.METRE.)
) ;
#24631=(
NAMED_UNIT(*)
PLANE_ANGLE_UNIT()
SI_UNIT($,.RADIAN.)
) ;
#24632=(
NAMED_UNIT(*)
SI_UNIT($,.STERADIAN.)
SOLID_ANGLE_UNIT()
) ;
#24657=SHAPE_DEFINITION_REPRESENTATION(#24726,#24815) ;
#24726=PRODUCT_DEFINITION_SHAPE('',$,#24863) ;
#24815=SHAPE_REPRESENTATION('',(#14884),#24605) ;
#24838=PRODUCT_DEFINITION_CONTEXT('part definition',#24981,'design') ;
#24863=PRODUCT_DEFINITION('FEED_ROLLER_HOUSING',
'FEED_ROLLER_HOUSING',#24910,#24838) ;
#24910=PRODUCT_DEFINITION_FORMATION('',$,#25007) ;
#24981=APPLICATION_CONTEXT(
'Core Data for Automotive Mechanical Design Process') ;
#24982=PRODUCT_CONTEXT('part definition',#24981,'mechanical') ;
#25007=PRODUCT('FEED_ROLLER_HOUSING','FEED_ROLLER_HOUSING',$,(#24982)) ;
#25031=PRESENTATION_STYLE_ASSIGNMENT((#25041)) ;
#25041=SURFACE_STYLE_USAGE(.BOTH.,#25051) ;
#25051=SURFACE_SIDE_STYLE('',(#25061)) ;
#25061=SURFACE_STYLE_FILL_AREA(#25071) ;
#25071=FILL_AREA_STYLE('Aluminum - Satin',(#25081)) ;
#25081=FILL_AREA_STYLE_COLOUR('Aluminum - Satin',#25091) ;
#25091=COLOUR_RGB('Aluminum - Satin', 0.40784314, 0.44705882, 0.49803922) ;
ENDSEC;
END-ISO-10303-21;
